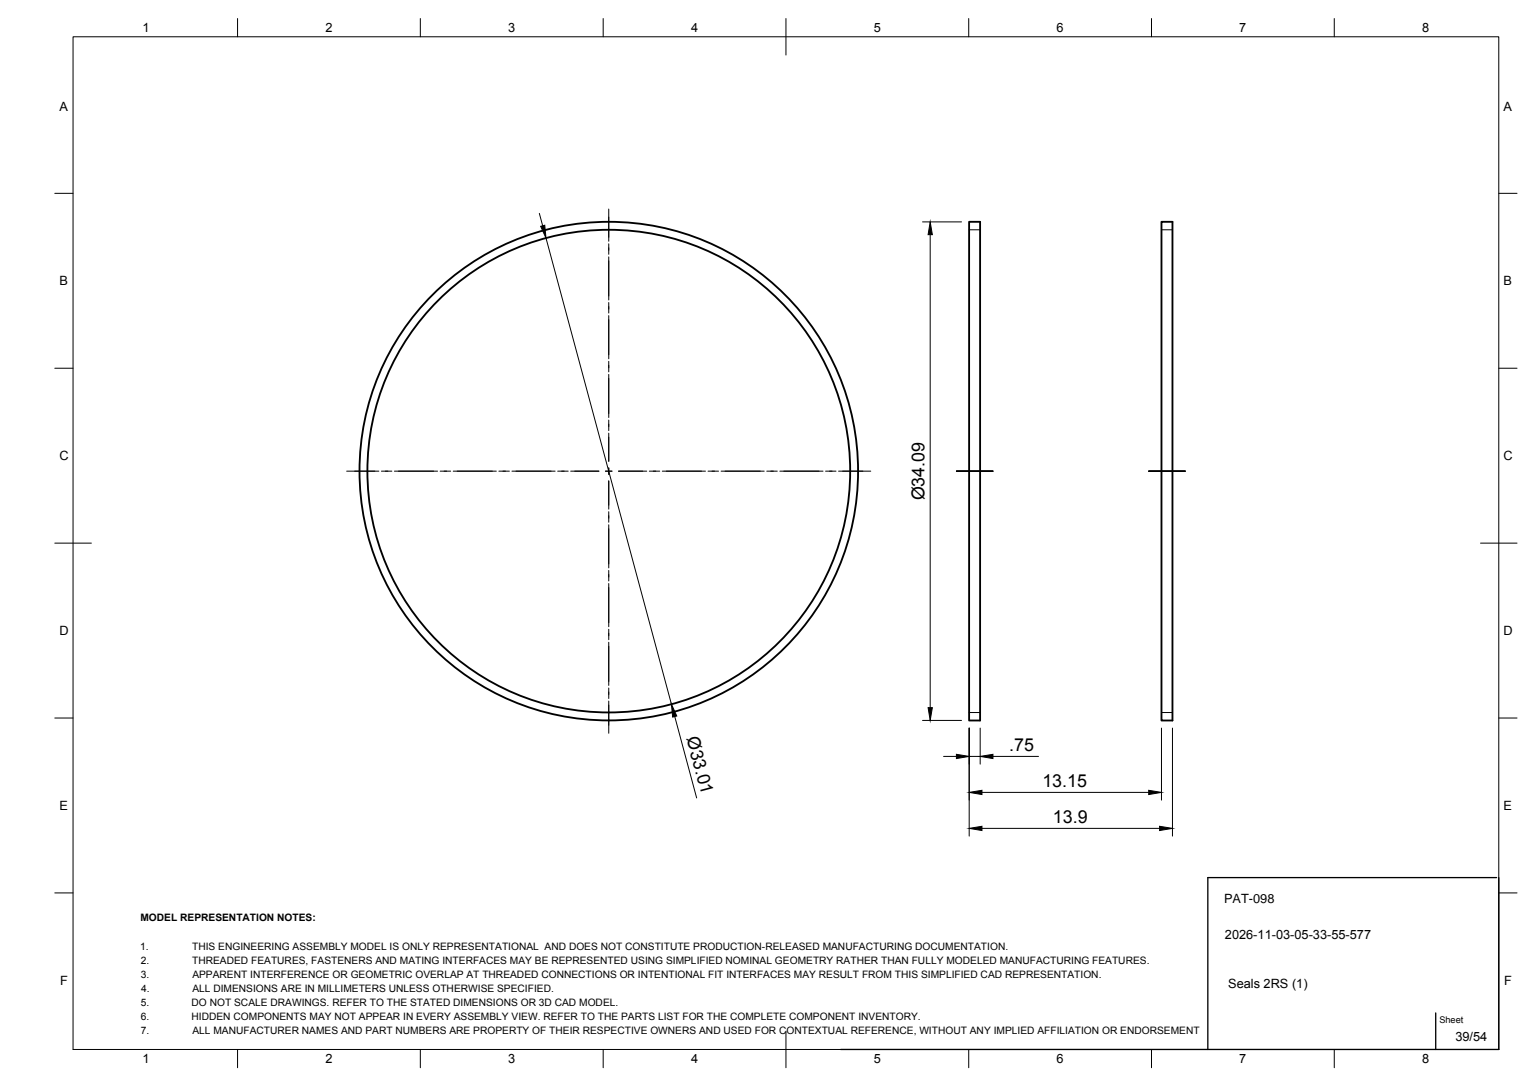
ISO-10303-21;
HEADER;
/* Generated by software containing ST-Developer
 * from STEP Tools, Inc. (www.steptools.com) 
 */

FILE_DESCRIPTION(
/* description */ ('Spring compression tester'),
/* implementation_level */ '2;1');

FILE_NAME(
/* name */ 'Seals 2RS (1).step',
/* time_stamp */ '2026-10-28T03:24:11-07:00',
/* author */ (''),
/* organization */ (''),
/* preprocessor_version */ 'ST-DEVELOPER v20.2',
/* originating_system */ 'Autodesk Translation Framework v15.17.0.0',
/* authorisation */ '');

FILE_SCHEMA (('AUTOMOTIVE_DESIGN { 1 0 10303 214 3 1 1 }'));
ENDSEC;

DATA;
#10=MECHANICAL_DESIGN_GEOMETRIC_PRESENTATION_REPRESENTATION('',(#1150,#1151),#43521);
#1016=SHAPE_REPRESENTATION_RELATIONSHIP('SRR','None',#43830,#1076);
#1076=ADVANCED_BREP_SHAPE_REPRESENTATION('',(#1224,#1225),#43490);
#1150=STYLED_ITEM('',(#44202),#1224);
#1151=STYLED_ITEM('',(#44202),#1225);
#1224=MANIFOLD_SOLID_BREP('Body1',#18588);
#1225=MANIFOLD_SOLID_BREP('Body2',#18589);
#1464=FACE_BOUND('',#3952,.T.);
#1465=FACE_BOUND('',#3955,.T.);
#1466=FACE_BOUND('',#3958,.T.);
#1467=FACE_BOUND('',#3961,.T.);
#1917=PLANE('',#20233);
#1918=PLANE('',#20238);
#1919=PLANE('',#20241);
#1920=PLANE('',#20246);
#2687=FACE_OUTER_BOUND('',#3951,.T.);
#2688=FACE_OUTER_BOUND('',#3953,.T.);
#2689=FACE_OUTER_BOUND('',#3954,.T.);
#2690=FACE_OUTER_BOUND('',#3956,.T.);
#2691=FACE_OUTER_BOUND('',#3957,.T.);
#2692=FACE_OUTER_BOUND('',#3959,.T.);
#2693=FACE_OUTER_BOUND('',#3960,.T.);
#2694=FACE_OUTER_BOUND('',#3962,.T.);
#3951=EDGE_LOOP('',(#14507));
#3952=EDGE_LOOP('',(#14508));
#3953=EDGE_LOOP('',(#14509,#14510,#14511,#14512));
#3954=EDGE_LOOP('',(#14513));
#3955=EDGE_LOOP('',(#14514));
#3956=EDGE_LOOP('',(#14515,#14516,#14517,#14518));
#3957=EDGE_LOOP('',(#14519));
#3958=EDGE_LOOP('',(#14520));
#3959=EDGE_LOOP('',(#14521,#14522,#14523,#14524));
#3960=EDGE_LOOP('',(#14525));
#3961=EDGE_LOOP('',(#14526));
#3962=EDGE_LOOP('',(#14527,#14528,#14529,#14530));
#5329=LINE('',#29575,#6761);
#5330=LINE('',#29580,#6762);
#5331=LINE('',#29589,#6763);
#5332=LINE('',#29594,#6764);
#6761=VECTOR('',#23827,1.70469);
#6762=VECTOR('',#23834,1.65031);
#6763=VECTOR('',#23845,1.70469);
#6764=VECTOR('',#23852,1.65031);
#7860=CIRCLE('',#20234,1.70469);
#7861=CIRCLE('',#20235,1.65031);
#7862=CIRCLE('',#20237,1.70469);
#7863=CIRCLE('',#20239,1.65031);
#7864=CIRCLE('',#20242,1.70469);
#7865=CIRCLE('',#20243,1.65031);
#7866=CIRCLE('',#20245,1.70469);
#7867=CIRCLE('',#20247,1.65031);
#8915=VERTEX_POINT('',#29568);
#8916=VERTEX_POINT('',#29570);
#8917=VERTEX_POINT('',#29573);
#8918=VERTEX_POINT('',#29577);
#8919=VERTEX_POINT('',#29582);
#8920=VERTEX_POINT('',#29584);
#8921=VERTEX_POINT('',#29587);
#8922=VERTEX_POINT('',#29591);
#10918=EDGE_CURVE('',#8915,#8915,#7860,.T.);
#10919=EDGE_CURVE('',#8916,#8916,#7861,.T.);
#10920=EDGE_CURVE('',#8917,#8917,#7862,.T.);
#10921=EDGE_CURVE('',#8917,#8915,#5329,.T.);
#10922=EDGE_CURVE('',#8918,#8918,#7863,.T.);
#10923=EDGE_CURVE('',#8918,#8916,#5330,.T.);
#10924=EDGE_CURVE('',#8919,#8919,#7864,.T.);
#10925=EDGE_CURVE('',#8920,#8920,#7865,.T.);
#10926=EDGE_CURVE('',#8921,#8921,#7866,.T.);
#10927=EDGE_CURVE('',#8921,#8919,#5331,.T.);
#10928=EDGE_CURVE('',#8922,#8922,#7867,.T.);
#10929=EDGE_CURVE('',#8922,#8920,#5332,.T.);
#14507=ORIENTED_EDGE('',*,*,#10918,.F.);
#14508=ORIENTED_EDGE('',*,*,#10919,.T.);
#14509=ORIENTED_EDGE('',*,*,#10920,.F.);
#14510=ORIENTED_EDGE('',*,*,#10921,.T.);
#14511=ORIENTED_EDGE('',*,*,#10918,.T.);
#14512=ORIENTED_EDGE('',*,*,#10921,.F.);
#14513=ORIENTED_EDGE('',*,*,#10920,.T.);
#14514=ORIENTED_EDGE('',*,*,#10922,.F.);
#14515=ORIENTED_EDGE('',*,*,#10922,.T.);
#14516=ORIENTED_EDGE('',*,*,#10923,.T.);
#14517=ORIENTED_EDGE('',*,*,#10919,.F.);
#14518=ORIENTED_EDGE('',*,*,#10923,.F.);
#14519=ORIENTED_EDGE('',*,*,#10924,.F.);
#14520=ORIENTED_EDGE('',*,*,#10925,.T.);
#14521=ORIENTED_EDGE('',*,*,#10926,.F.);
#14522=ORIENTED_EDGE('',*,*,#10927,.T.);
#14523=ORIENTED_EDGE('',*,*,#10924,.T.);
#14524=ORIENTED_EDGE('',*,*,#10927,.F.);
#14525=ORIENTED_EDGE('',*,*,#10926,.T.);
#14526=ORIENTED_EDGE('',*,*,#10928,.F.);
#14527=ORIENTED_EDGE('',*,*,#10928,.T.);
#14528=ORIENTED_EDGE('',*,*,#10929,.T.);
#14529=ORIENTED_EDGE('',*,*,#10925,.F.);
#14530=ORIENTED_EDGE('',*,*,#10929,.F.);
#17247=CYLINDRICAL_SURFACE('',#20236,1.70469);
#17248=CYLINDRICAL_SURFACE('',#20240,1.65031);
#17249=CYLINDRICAL_SURFACE('',#20244,1.70469);
#17250=CYLINDRICAL_SURFACE('',#20248,1.65031);
#18011=ADVANCED_FACE('',(#2687,#1464),#1917,.T.);
#18012=ADVANCED_FACE('',(#2688),#17247,.T.);
#18013=ADVANCED_FACE('',(#2689,#1465),#1918,.T.);
#18014=ADVANCED_FACE('',(#2690),#17248,.F.);
#18015=ADVANCED_FACE('',(#2691,#1466),#1919,.T.);
#18016=ADVANCED_FACE('',(#2692),#17249,.T.);
#18017=ADVANCED_FACE('',(#2693,#1467),#1920,.T.);
#18018=ADVANCED_FACE('',(#2694),#17250,.F.);
#18588=CLOSED_SHELL('',(#18011,#18012,#18013,#18014));
#18589=CLOSED_SHELL('',(#18015,#18016,#18017,#18018));
#20232=AXIS2_PLACEMENT_3D('',#29566,#23815,#23816);
#20233=AXIS2_PLACEMENT_3D('',#29567,#23817,#23818);
#20234=AXIS2_PLACEMENT_3D('',#29569,#23819,#23820);
#20235=AXIS2_PLACEMENT_3D('',#29571,#23821,#23822);
#20236=AXIS2_PLACEMENT_3D('',#29572,#23823,#23824);
#20237=AXIS2_PLACEMENT_3D('',#29574,#23825,#23826);
#20238=AXIS2_PLACEMENT_3D('',#29576,#23828,#23829);
#20239=AXIS2_PLACEMENT_3D('',#29578,#23830,#23831);
#20240=AXIS2_PLACEMENT_3D('',#29579,#23832,#23833);
#20241=AXIS2_PLACEMENT_3D('',#29581,#23835,#23836);
#20242=AXIS2_PLACEMENT_3D('',#29583,#23837,#23838);
#20243=AXIS2_PLACEMENT_3D('',#29585,#23839,#23840);
#20244=AXIS2_PLACEMENT_3D('',#29586,#23841,#23842);
#20245=AXIS2_PLACEMENT_3D('',#29588,#23843,#23844);
#20246=AXIS2_PLACEMENT_3D('',#29590,#23846,#23847);
#20247=AXIS2_PLACEMENT_3D('',#29592,#23848,#23849);
#20248=AXIS2_PLACEMENT_3D('',#29593,#23850,#23851);
#23815=DIRECTION('axis',(0.,0.,1.));
#23816=DIRECTION('refdir',(1.,0.,0.));
#23817=DIRECTION('center_axis',(0.,1.,0.));
#23818=DIRECTION('ref_axis',(0.,0.,1.));
#23819=DIRECTION('center_axis',(0.,-1.,0.));
#23820=DIRECTION('ref_axis',(1.,0.,0.));
#23821=DIRECTION('center_axis',(0.,-1.,0.));
#23822=DIRECTION('ref_axis',(1.,0.,0.));
#23823=DIRECTION('center_axis',(0.,-1.,0.));
#23824=DIRECTION('ref_axis',(1.,0.,0.));
#23825=DIRECTION('center_axis',(0.,-1.,0.));
#23826=DIRECTION('ref_axis',(1.,0.,0.));
#23827=DIRECTION('',(0.,1.,0.));
#23828=DIRECTION('center_axis',(0.,-1.,0.));
#23829=DIRECTION('ref_axis',(0.,0.,-1.));
#23830=DIRECTION('center_axis',(0.,-1.,0.));
#23831=DIRECTION('ref_axis',(1.,0.,0.));
#23832=DIRECTION('center_axis',(0.,-1.,0.));
#23833=DIRECTION('ref_axis',(1.,0.,0.));
#23834=DIRECTION('',(0.,1.,0.));
#23835=DIRECTION('center_axis',(0.,1.,0.));
#23836=DIRECTION('ref_axis',(0.,0.,1.));
#23837=DIRECTION('center_axis',(0.,-1.,0.));
#23838=DIRECTION('ref_axis',(1.,0.,0.));
#23839=DIRECTION('center_axis',(0.,-1.,0.));
#23840=DIRECTION('ref_axis',(1.,0.,0.));
#23841=DIRECTION('center_axis',(0.,-1.,0.));
#23842=DIRECTION('ref_axis',(1.,0.,0.));
#23843=DIRECTION('center_axis',(0.,-1.,0.));
#23844=DIRECTION('ref_axis',(1.,0.,0.));
#23845=DIRECTION('',(0.,1.,0.));
#23846=DIRECTION('center_axis',(0.,-1.,0.));
#23847=DIRECTION('ref_axis',(0.,0.,-1.));
#23848=DIRECTION('center_axis',(0.,-1.,0.));
#23849=DIRECTION('ref_axis',(1.,0.,0.));
#23850=DIRECTION('center_axis',(0.,-1.,0.));
#23851=DIRECTION('ref_axis',(1.,0.,0.));
#23852=DIRECTION('',(0.,1.,0.));
#29566=CARTESIAN_POINT('',(0.,0.,0.));
#29567=CARTESIAN_POINT('Origin',(1.70469,0.695,0.));
#29568=CARTESIAN_POINT('',(-1.70469,0.695,-2.0876431520385E-16));
#29569=CARTESIAN_POINT('Origin',(0.,0.695,0.));
#29570=CARTESIAN_POINT('',(-1.65031,0.695,-2.02104685910087E-16));
#29571=CARTESIAN_POINT('Origin',(0.,0.695,0.));
#29572=CARTESIAN_POINT('Origin',(0.,0.6575,0.));
#29573=CARTESIAN_POINT('',(-1.70469,0.62,-2.0876431520385E-16));
#29574=CARTESIAN_POINT('Origin',(0.,0.62,0.));
#29575=CARTESIAN_POINT('',(-1.70469,0.6575,-2.0876431520385E-16));
#29576=CARTESIAN_POINT('Origin',(1.65031,0.62,0.));
#29577=CARTESIAN_POINT('',(-1.65031,0.62,-2.02104685910087E-16));
#29578=CARTESIAN_POINT('Origin',(0.,0.62,0.));
#29579=CARTESIAN_POINT('Origin',(0.,0.6575,0.));
#29580=CARTESIAN_POINT('',(-1.65031,0.6575,-2.02104685910087E-16));
#29581=CARTESIAN_POINT('Origin',(1.70469,-0.62,0.));
#29582=CARTESIAN_POINT('',(-1.70469,-0.62,-2.0876431520385E-16));
#29583=CARTESIAN_POINT('Origin',(0.,-0.62,0.));
#29584=CARTESIAN_POINT('',(-1.65031,-0.62,-2.02104685910087E-16));
#29585=CARTESIAN_POINT('Origin',(0.,-0.62,0.));
#29586=CARTESIAN_POINT('Origin',(0.,-0.6575,0.));
#29587=CARTESIAN_POINT('',(-1.70469,-0.695,-2.0876431520385E-16));
#29588=CARTESIAN_POINT('Origin',(0.,-0.695,0.));
#29589=CARTESIAN_POINT('',(-1.70469,-0.6575,-2.0876431520385E-16));
#29590=CARTESIAN_POINT('Origin',(1.65031,-0.695,0.));
#29591=CARTESIAN_POINT('',(-1.65031,-0.695,-2.02104685910087E-16));
#29592=CARTESIAN_POINT('Origin',(0.,-0.695,0.));
#29593=CARTESIAN_POINT('Origin',(0.,-0.6575,0.));
#29594=CARTESIAN_POINT('',(-1.65031,-0.6575,-2.02104685910087E-16));
#43422=UNCERTAINTY_MEASURE_WITH_UNIT(LENGTH_MEASURE(0.001),#43522,
'DISTANCE_ACCURACY_VALUE',
'Maximum model space distance between geometric entities at asserted c
onnectivities');
#43453=UNCERTAINTY_MEASURE_WITH_UNIT(LENGTH_MEASURE(0.001),#43522,
'DISTANCE_ACCURACY_VALUE',
'Maximum model space distance between geometric entities at asserted c
onnectivities');
#43490=(
GEOMETRIC_REPRESENTATION_CONTEXT(3)
GLOBAL_UNCERTAINTY_ASSIGNED_CONTEXT((#43422))
GLOBAL_UNIT_ASSIGNED_CONTEXT((#43522,#43524,#43525))
REPRESENTATION_CONTEXT('','3D')
);
#43521=(
GEOMETRIC_REPRESENTATION_CONTEXT(3)
GLOBAL_UNCERTAINTY_ASSIGNED_CONTEXT((#43453))
GLOBAL_UNIT_ASSIGNED_CONTEXT((#43522,#43524,#43525))
REPRESENTATION_CONTEXT('','3D')
);
#43522=(
LENGTH_UNIT()
NAMED_UNIT(*)
SI_UNIT(.CENTI.,.METRE.)
);
#43524=(
NAMED_UNIT(*)
PLANE_ANGLE_UNIT()
SI_UNIT($,.RADIAN.)
);
#43525=(
NAMED_UNIT(*)
SI_UNIT($,.STERADIAN.)
SOLID_ANGLE_UNIT()
);
#43562=SHAPE_DEFINITION_REPRESENTATION(#43634,#43830);
#43634=PRODUCT_DEFINITION_SHAPE('',$,#43898);
#43830=SHAPE_REPRESENTATION('',(#20232),#43490);
#43861=PRODUCT_DEFINITION_CONTEXT('part definition',#44064,'design');
#43898=PRODUCT_DEFINITION('Seals 2RS (1)','Seals 2RS (1)',#43965,#43861);
#43965=PRODUCT_DEFINITION_FORMATION('',$,#44102);
#44064=APPLICATION_CONTEXT(
'Core Data for Automotive Mechanical Design Process');
#44065=PRODUCT_CONTEXT('part definition',#44064,'mechanical');
#44102=PRODUCT('Seals 2RS (1)','Seals 2RS (1)','Seals 2RS (1)',(#44065));
#44196=COLOUR_RGB('Grey',0.48,0.52,0.57);
#44197=FILL_AREA_STYLE_COLOUR('',#44196);
#44198=FILL_AREA_STYLE('',(#44197));
#44199=SURFACE_STYLE_FILL_AREA(#44198);
#44200=SURFACE_SIDE_STYLE('',(#44199));
#44201=SURFACE_STYLE_USAGE(.BOTH.,#44200);
#44202=PRESENTATION_STYLE_ASSIGNMENT((#44201));
ENDSEC;
END-ISO-10303-21;
